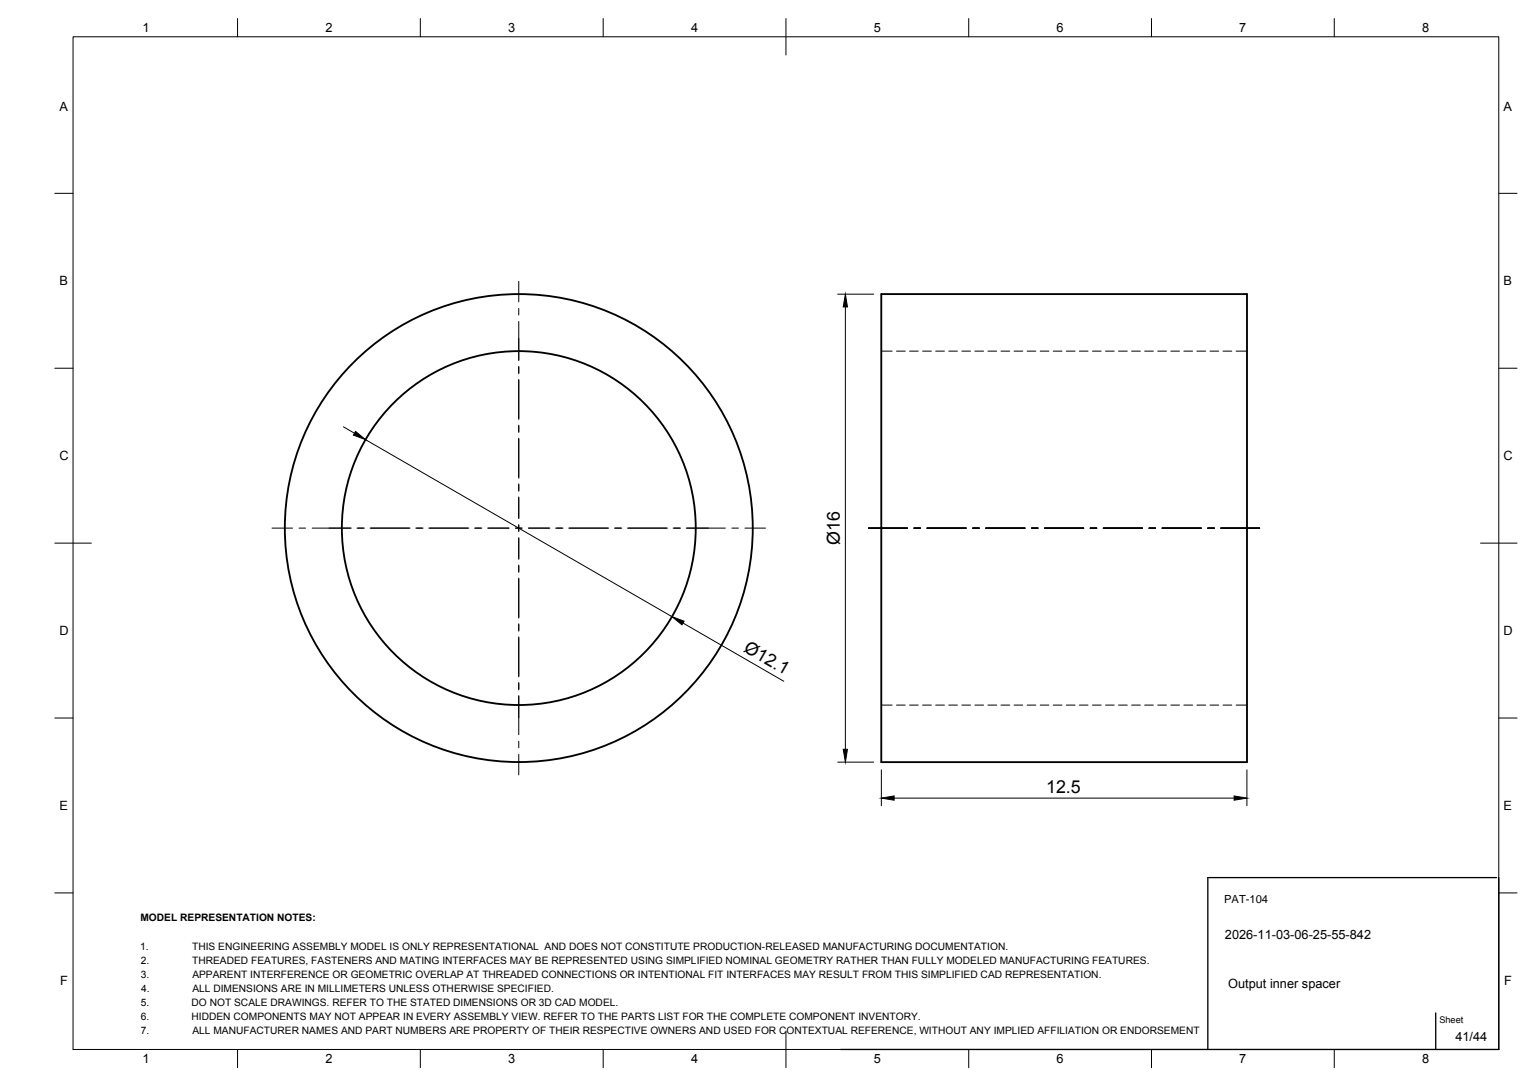
ISO-10303-21;
HEADER;
/* Generated by software containing ST-Developer
 * from STEP Tools, Inc. (www.steptools.com) 
 */

FILE_DESCRIPTION(
/* description */ ('Timing belt drive module 2 mm Pitch Timing 20T-40T'),

/* implementation_level */ '2;1');

FILE_NAME(
/* name */ 'Output inner spacer.step',
/* time_stamp */ '2026-10-28T03:25:12-07:00',
/* author */ (''),
/* organization */ (''),
/* preprocessor_version */ 'ST-DEVELOPER v20.2',
/* originating_system */ 'Autodesk Translation Framework v15.17.0.0',
/* authorisation */ '');

FILE_SCHEMA (('AUTOMOTIVE_DESIGN { 1 0 10303 214 3 1 1 }'));
ENDSEC;

DATA;
#10=MECHANICAL_DESIGN_GEOMETRIC_PRESENTATION_REPRESENTATION('',(#575),#17830);
#474=SHAPE_REPRESENTATION_RELATIONSHIP('SRR','None',#18048,#517);
#517=ADVANCED_BREP_SHAPE_REPRESENTATION('',(#631),#17823);
#575=STYLED_ITEM('',(#18310),#631);
#631=MANIFOLD_SOLID_BREP('Body1',#9034);
#755=FACE_BOUND('',#1997,.T.);
#756=FACE_BOUND('',#1999,.T.);
#936=PLANE('',#10426);
#937=PLANE('',#10427);
#1355=FACE_OUTER_BOUND('',#1994,.T.);
#1356=FACE_OUTER_BOUND('',#1995,.T.);
#1357=FACE_OUTER_BOUND('',#1996,.T.);
#1358=FACE_OUTER_BOUND('',#1998,.T.);
#1994=EDGE_LOOP('',(#7509,#7510,#7511,#7512));
#1995=EDGE_LOOP('',(#7513,#7514,#7515,#7516));
#1996=EDGE_LOOP('',(#7517));
#1997=EDGE_LOOP('',(#7518));
#1998=EDGE_LOOP('',(#7519));
#1999=EDGE_LOOP('',(#7520));
#2598=CIRCLE('',#10421,0.605);
#2599=CIRCLE('',#10422,0.605);
#2600=CIRCLE('',#10424,0.8);
#2601=CIRCLE('',#10425,0.8);
#3146=LINE('',#16698,#3624);
#3147=LINE('',#16704,#3625);
#3624=VECTOR('',#12977,0.605);
#3625=VECTOR('',#12984,0.8);
#4343=VERTEX_POINT('',#16695);
#4344=VERTEX_POINT('',#16697);
#4345=VERTEX_POINT('',#16701);
#4346=VERTEX_POINT('',#16703);
#5437=EDGE_CURVE('',#4343,#4343,#2598,.T.);
#5438=EDGE_CURVE('',#4343,#4344,#3146,.T.);
#5439=EDGE_CURVE('',#4344,#4344,#2599,.T.);
#5440=EDGE_CURVE('',#4345,#4345,#2600,.T.);
#5441=EDGE_CURVE('',#4345,#4346,#3147,.T.);
#5442=EDGE_CURVE('',#4346,#4346,#2601,.T.);
#7509=ORIENTED_EDGE('',*,*,#5437,.F.);
#7510=ORIENTED_EDGE('',*,*,#5438,.T.);
#7511=ORIENTED_EDGE('',*,*,#5439,.T.);
#7512=ORIENTED_EDGE('',*,*,#5438,.F.);
#7513=ORIENTED_EDGE('',*,*,#5440,.F.);
#7514=ORIENTED_EDGE('',*,*,#5441,.T.);
#7515=ORIENTED_EDGE('',*,*,#5442,.T.);
#7516=ORIENTED_EDGE('',*,*,#5441,.F.);
#7517=ORIENTED_EDGE('',*,*,#5440,.T.);
#7518=ORIENTED_EDGE('',*,*,#5437,.T.);
#7519=ORIENTED_EDGE('',*,*,#5442,.F.);
#7520=ORIENTED_EDGE('',*,*,#5439,.F.);
#8362=CYLINDRICAL_SURFACE('',#10420,0.605);
#8363=CYLINDRICAL_SURFACE('',#10423,0.8);
#8853=ADVANCED_FACE('',(#1355),#8362,.F.);
#8854=ADVANCED_FACE('',(#1356),#8363,.T.);
#8855=ADVANCED_FACE('',(#1357,#755),#936,.T.);
#8856=ADVANCED_FACE('',(#1358,#756),#937,.F.);
#9034=CLOSED_SHELL('',(#8853,#8854,#8855,#8856));
#10419=AXIS2_PLACEMENT_3D('',#16693,#12971,#12972);
#10420=AXIS2_PLACEMENT_3D('',#16694,#12973,#12974);
#10421=AXIS2_PLACEMENT_3D('',#16696,#12975,#12976);
#10422=AXIS2_PLACEMENT_3D('',#16699,#12978,#12979);
#10423=AXIS2_PLACEMENT_3D('',#16700,#12980,#12981);
#10424=AXIS2_PLACEMENT_3D('',#16702,#12982,#12983);
#10425=AXIS2_PLACEMENT_3D('',#16705,#12985,#12986);
#10426=AXIS2_PLACEMENT_3D('',#16706,#12987,#12988);
#10427=AXIS2_PLACEMENT_3D('',#16707,#12989,#12990);
#12971=DIRECTION('axis',(0.,0.,1.));
#12972=DIRECTION('refdir',(1.,0.,0.));
#12973=DIRECTION('center_axis',(0.,1.,0.));
#12974=DIRECTION('ref_axis',(1.,0.,0.));
#12975=DIRECTION('center_axis',(0.,-1.,0.));
#12976=DIRECTION('ref_axis',(1.,0.,0.));
#12977=DIRECTION('',(0.,-1.,0.));
#12978=DIRECTION('center_axis',(0.,-1.,0.));
#12979=DIRECTION('ref_axis',(1.,0.,0.));
#12980=DIRECTION('center_axis',(0.,1.,0.));
#12981=DIRECTION('ref_axis',(1.,0.,0.));
#12982=DIRECTION('center_axis',(0.,1.,0.));
#12983=DIRECTION('ref_axis',(1.,0.,0.));
#12984=DIRECTION('',(0.,-1.,0.));
#12985=DIRECTION('center_axis',(0.,1.,0.));
#12986=DIRECTION('ref_axis',(1.,0.,0.));
#12987=DIRECTION('center_axis',(0.,1.,0.));
#12988=DIRECTION('ref_axis',(1.,0.,0.));
#12989=DIRECTION('center_axis',(0.,1.,0.));
#12990=DIRECTION('ref_axis',(1.,0.,0.));
#16693=CARTESIAN_POINT('',(0.,0.,0.));
#16694=CARTESIAN_POINT('Origin',(6.97091003018116,-2.65,7.));
#16695=CARTESIAN_POINT('',(6.36591003018116,-1.4,7.));
#16696=CARTESIAN_POINT('Origin',(6.97091003018116,-1.4,7.));
#16697=CARTESIAN_POINT('',(6.36591003018116,-2.65,7.));
#16698=CARTESIAN_POINT('',(6.36591003018116,-2.65,7.));
#16699=CARTESIAN_POINT('Origin',(6.97091003018116,-2.65,7.));
#16700=CARTESIAN_POINT('Origin',(6.97091003018116,-2.65,7.));
#16701=CARTESIAN_POINT('',(6.17091003018116,-1.4,7.));
#16702=CARTESIAN_POINT('Origin',(6.97091003018116,-1.4,7.));
#16703=CARTESIAN_POINT('',(6.17091003018116,-2.65,7.));
#16704=CARTESIAN_POINT('',(6.17091003018116,-2.65,7.));
#16705=CARTESIAN_POINT('Origin',(6.97091003018116,-2.65,7.));
#16706=CARTESIAN_POINT('Origin',(6.97091003018116,-1.4,7.));
#16707=CARTESIAN_POINT('Origin',(6.97091003018116,-2.65,7.));
#17773=UNCERTAINTY_MEASURE_WITH_UNIT(LENGTH_MEASURE(0.001),#17831,
'DISTANCE_ACCURACY_VALUE',
'Maximum model space distance between geometric entities at asserted c
onnectivities');
#17780=UNCERTAINTY_MEASURE_WITH_UNIT(LENGTH_MEASURE(0.001),#17831,
'DISTANCE_ACCURACY_VALUE',
'Maximum model space distance between geometric entities at asserted c
onnectivities');
#17823=(
GEOMETRIC_REPRESENTATION_CONTEXT(3)
GLOBAL_UNCERTAINTY_ASSIGNED_CONTEXT((#17773))
GLOBAL_UNIT_ASSIGNED_CONTEXT((#17831,#17833,#17834))
REPRESENTATION_CONTEXT('','3D')
);
#17830=(
GEOMETRIC_REPRESENTATION_CONTEXT(3)
GLOBAL_UNCERTAINTY_ASSIGNED_CONTEXT((#17780))
GLOBAL_UNIT_ASSIGNED_CONTEXT((#17831,#17833,#17834))
REPRESENTATION_CONTEXT('','3D')
);
#17831=(
LENGTH_UNIT()
NAMED_UNIT(*)
SI_UNIT(.CENTI.,.METRE.)
);
#17833=(
NAMED_UNIT(*)
PLANE_ANGLE_UNIT()
SI_UNIT($,.RADIAN.)
);
#17834=(
NAMED_UNIT(*)
SI_UNIT($,.STERADIAN.)
SOLID_ANGLE_UNIT()
);
#17877=SHAPE_DEFINITION_REPRESENTATION(#17936,#18048);
#17936=PRODUCT_DEFINITION_SHAPE('',$,#18098);
#18048=SHAPE_REPRESENTATION('',(#10419),#17823);
#18055=PRODUCT_DEFINITION_CONTEXT('part definition',#18204,'design');
#18098=PRODUCT_DEFINITION('Output inner spacer','Output inner spacer',#18147,
#18055);
#18147=PRODUCT_DEFINITION_FORMATION('',$,#18248);
#18204=APPLICATION_CONTEXT(
'Core Data for Automotive Mechanical Design Process');
#18205=PRODUCT_CONTEXT('part definition',#18204,'mechanical');
#18248=PRODUCT('Output inner spacer','Output inner spacer',
'Output inner spacer',(#18205));
#18304=COLOUR_RGB('Sky Blue',0.24,0.69,0.87);
#18305=FILL_AREA_STYLE_COLOUR('',#18304);
#18306=FILL_AREA_STYLE('',(#18305));
#18307=SURFACE_STYLE_FILL_AREA(#18306);
#18308=SURFACE_SIDE_STYLE('',(#18307));
#18309=SURFACE_STYLE_USAGE(.BOTH.,#18308);
#18310=PRESENTATION_STYLE_ASSIGNMENT((#18309));
ENDSEC;
END-ISO-10303-21;
